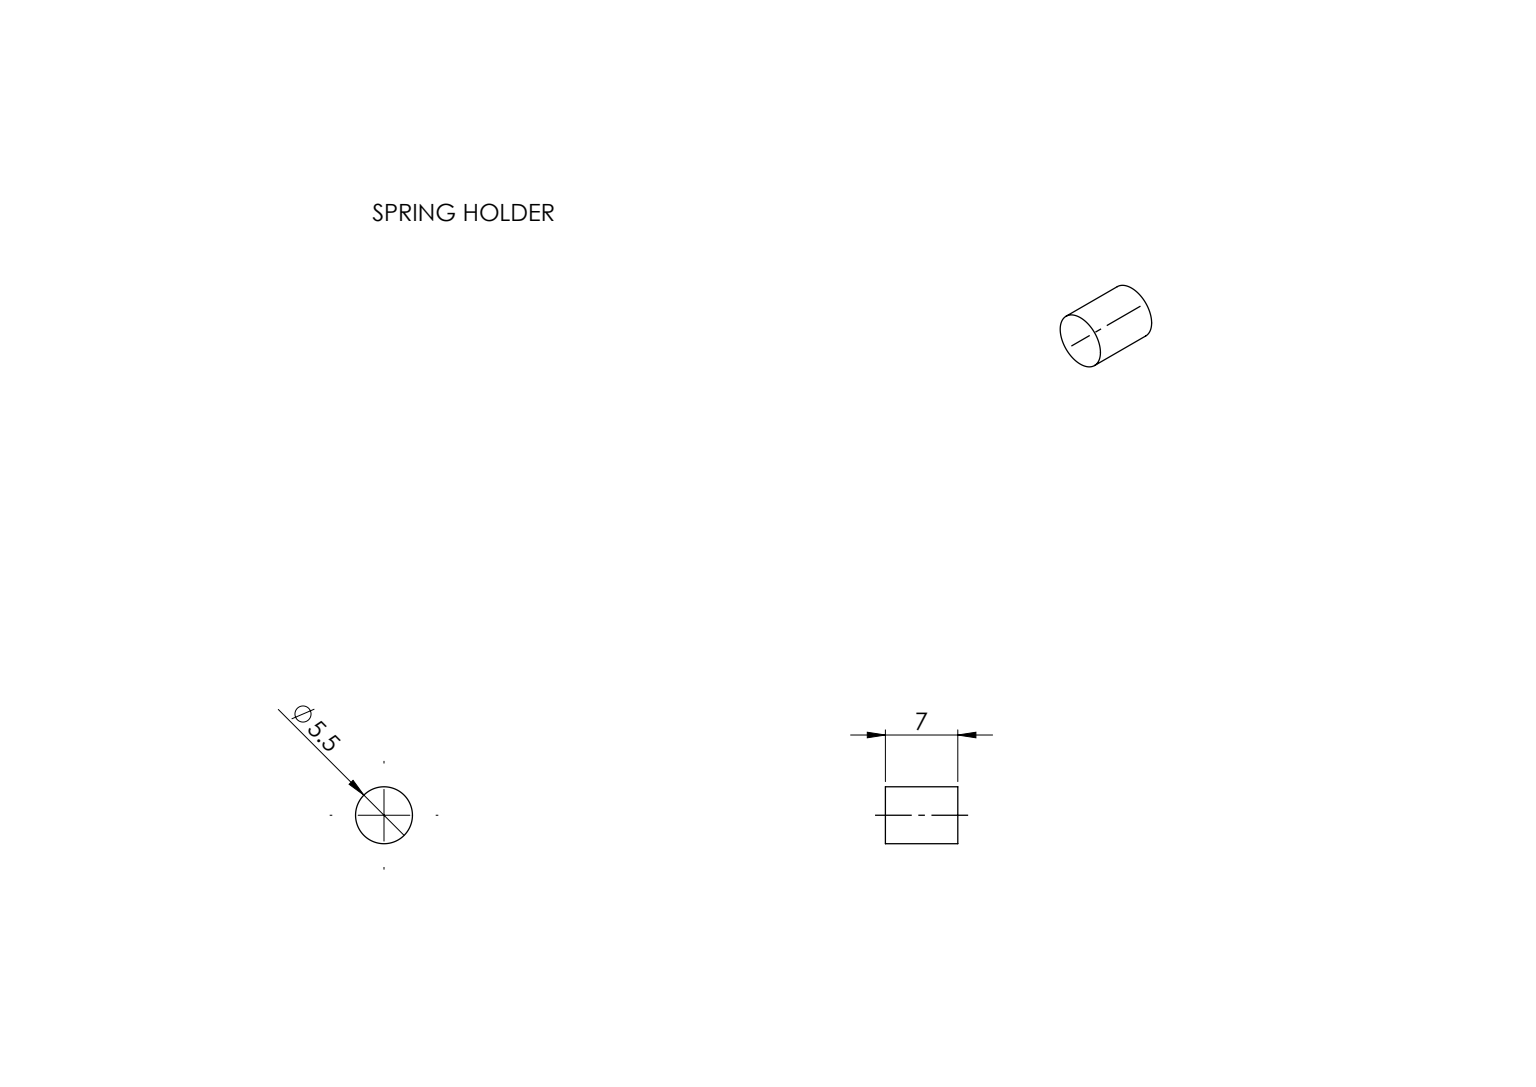
ISO-10303-21;
HEADER;
FILE_DESCRIPTION (('STEP AP214'),
    '1' );
FILE_NAME ('spring holder.step',
    '2026-10-05T05:16:24',
    ( '' ),
    ( '' ),
    'SwSTEP 2.0',
    'SolidWorks 2026',
    '' );
FILE_SCHEMA (( 'AUTOMOTIVE_DESIGN' ));
ENDSEC;

DATA;
#534=CARTESIAN_POINT ( 'NONE',  ( 1.653273178848927064E-15, -7.500000000000000000, 11.00000000000000178 ) ) ;
#1888=MECHANICAL_DESIGN_GEOMETRIC_PRESENTATION_REPRESENTATION('',(#79567),#65141);
#2272=UNCERTAINTY_MEASURE_WITH_UNIT (LENGTH_MEASURE( 1.000000000000000082E-05 ), #31200, 'distance_accuracy_value', 'NONE');
#3063=VERTEX_POINT ( 'NONE', #51324 ) ;
#4174=( LENGTH_UNIT ( ) NAMED_UNIT ( * ) SI_UNIT ( .MILLI., .METRE. ) );
#4325=VERTEX_POINT ( 'NONE', #12504 ) ;
#7485=DIRECTION ( 'NONE',  ( 1.000000000000000000, 0.000000000000000000, -0.000000000000000000 ) ) ;
#8165=AXIS2_PLACEMENT_3D ( 'NONE', #19814, #47277, #40542 ) ;
#8975=CARTESIAN_POINT ( 'NONE',  ( 1.653273178848927064E-15, -7.500000000000000000, 11.00000000000000178 ) ) ;
#9438=DIRECTION ( 'NONE',  ( 0.000000000000000000, 0.000000000000000000, 1.000000000000000000 ) ) ;
#10500=( NAMED_UNIT ( * ) SI_UNIT ( $, .STERADIAN. ) SOLID_ANGLE_UNIT ( ) );
#10751=VERTEX_POINT ( 'NONE', #18242 ) ;
#11381=( NAMED_UNIT ( * ) SI_UNIT ( $, .STERADIAN. ) SOLID_ANGLE_UNIT ( ) );
#11508=ORIENTED_EDGE ( 'NONE', *, *, #70839, .F. ) ;
#11527=SHAPE_REPRESENTATION ( 'spring holder', ( #83448 ), #56118 ) ;
#11836=FILL_AREA_STYLE ('',( #72187 ) ) ;
#12321=DIRECTION ( 'NONE',  ( 1.000000000000000000, 0.000000000000000000, -0.000000000000000000 ) ) ;
#12504=CARTESIAN_POINT ( 'NONE',  ( 2.750000000000001776, -7.500000000000000000, 11.00000000000000178 ) ) ;
#13007=APPLICATION_CONTEXT ( 'automotive_design' ) ;
#13034=CIRCLE ( 'NONE', #79184, 2.750000000000000000 ) ;
#13162=DIRECTION ( 'NONE',  ( 0.000000000000000000, 0.000000000000000000, 1.000000000000000000 ) ) ;
#13210=EDGE_LOOP ( 'NONE', ( #17041, #44560, #75203, #61413 ) ) ;
#14259=CARTESIAN_POINT ( 'NONE',  ( -2.749999999999998224, -7.500000000000000000, 11.00000000000000178 ) ) ;
#15733=DIRECTION ( 'NONE',  ( 0.000000000000000000, 0.000000000000000000, 1.000000000000000000 ) ) ;
#15761=DIRECTION ( 'NONE',  ( 1.000000000000000000, 0.000000000000000000, 0.000000000000000000 ) ) ;
#16170=DIRECTION ( 'NONE',  ( 0.000000000000000000, 0.000000000000000000, 1.000000000000000000 ) ) ;
#16194=CARTESIAN_POINT ( 'NONE',  ( 1.653273178848927064E-15, -7.500000000000000000, 11.00000000000000178 ) ) ;
#16800=PRESENTATION_STYLE_ASSIGNMENT (( #37969 ) ) ;
#17041=ORIENTED_EDGE ( 'NONE', *, *, #71531, .T. ) ;
#17272=COLOUR_RGB ( '', 0.66274510, 0.83137255, 0.94901961) ;
#17657=VECTOR ( 'NONE', #15733, 1000.000000000000000 ) ;
#18242=CARTESIAN_POINT ( 'NONE',  ( 2.750000000000001776, -7.500000000000000000, 18.00000000000000355 ) ) ;
#19513=CARTESIAN_POINT ( 'NONE',  ( 1.653273178848927064E-15, -7.500000000000000000, 11.00000000000000178 ) ) ;
#19678=ADVANCED_FACE ( 'NONE', ( #57151 ), #77863, .T. ) ;
#19814=CARTESIAN_POINT ( 'NONE',  ( 1.653273178848927064E-15, -7.500000000000000000, 11.00000000000000178 ) ) ;
#19995=PRODUCT_DEFINITION ( 'UNKNOWN', '', #54748, #85206 ) ;
#23003=( GEOMETRIC_REPRESENTATION_CONTEXT ( 3 ) GLOBAL_UNCERTAINTY_ASSIGNED_CONTEXT ( ( #2272 ) ) GLOBAL_UNIT_ASSIGNED_CONTEXT ( ( #31200, #65434, #11381 ) ) REPRESENTATION_CONTEXT ( 'NONE', 'WORKASPACE' ) );
#23878=ORIENTED_EDGE ( 'NONE', *, *, #58802, .T. ) ;
#24904=COLOUR_RGB ( '', 0.66274510, 0.83137255, 0.94901961) ;
#26814=SURFACE_STYLE_USAGE ( .BOTH. , #33125 ) ;
#26851=DIRECTION ( 'NONE',  ( 0.000000000000000000, 0.000000000000000000, 1.000000000000000000 ) ) ;
#28181=DIRECTION ( 'NONE',  ( 0.000000000000000000, 0.000000000000000000, 1.000000000000000000 ) ) ;
#29592=AXIS2_PLACEMENT_3D ( 'NONE', #61073, #26851, #60180 ) ;
#30303=ORIENTED_EDGE ( 'NONE', *, *, #35419, .T. ) ;
#31200=( LENGTH_UNIT ( ) NAMED_UNIT ( * ) SI_UNIT ( .MILLI., .METRE. ) );
#31566=EDGE_LOOP ( 'NONE', ( #79815, #45791 ) ) ;
#32575=AXIS2_PLACEMENT_3D ( 'NONE', #534, #13162, #80749 ) ;
#32871=VERTEX_POINT ( 'NONE', #59707 ) ;
#33125=SURFACE_SIDE_STYLE ('',( #61472 ) ) ;
#34939=PLANE ( 'NONE',  #68533 ) ;
#35307=DIRECTION ( 'NONE',  ( 1.000000000000000000, 0.000000000000000000, 0.000000000000000000 ) ) ;
#35419=EDGE_CURVE ( 'NONE', #10751, #3063, #72731, .T. ) ;
#35562=LINE ( 'NONE', #77424, #17657 ) ;
#36528=UNCERTAINTY_MEASURE_WITH_UNIT (LENGTH_MEASURE( 1.000000000000000082E-05 ), #4174, 'distance_accuracy_value', 'NONE');
#37969=SURFACE_STYLE_USAGE ( .BOTH. , #53246 ) ;
#39006=ADVANCED_FACE ( 'NONE', ( #60940 ), #74026, .F. ) ;
#39898=PRESENTATION_STYLE_ASSIGNMENT (( #26814 ) ) ;
#40542=DIRECTION ( 'NONE',  ( 1.000000000000000000, 0.000000000000000000, 0.000000000000000000 ) ) ;
#40780=( NAMED_UNIT ( * ) SI_UNIT ( $, .STERADIAN. ) SOLID_ANGLE_UNIT ( ) );
#40850=LINE ( 'NONE', #14259, #69938 ) ;
#41724=MECHANICAL_DESIGN_GEOMETRIC_PRESENTATION_REPRESENTATION('',(#80559),#23003);
#43632=DIRECTION ( 'NONE',  ( 1.000000000000000000, 0.000000000000000000, 0.000000000000000000 ) ) ;
#44254=( NAMED_UNIT ( * ) PLANE_ANGLE_UNIT ( ) SI_UNIT ( $, .RADIAN. ) );
#44325=CLOSED_SHELL ( 'NONE', ( #19678, #71875, #39006, #63524 ) ) ;
#44560=ORIENTED_EDGE ( 'NONE', *, *, #70839, .T. ) ;
#44894=ORIENTED_EDGE ( 'NONE', *, *, #81635, .T. ) ;
#45791=ORIENTED_EDGE ( 'NONE', *, *, #81635, .F. ) ;
#46002=PRODUCT_CONTEXT ( 'NONE', #13007, 'mechanical' ) ;
#46452=CIRCLE ( 'NONE', #85289, 2.750000000000000000 ) ;
#47277=DIRECTION ( 'NONE',  ( 0.000000000000000000, 0.000000000000000000, 1.000000000000000000 ) ) ;
#48901=CARTESIAN_POINT ( 'NONE',  ( 1.653273178848927064E-15, -7.500000000000000000, 18.00000000000000355 ) ) ;
#51324=CARTESIAN_POINT ( 'NONE',  ( -2.749999999999998224, -7.500000000000000000, 18.00000000000000355 ) ) ;
#53246=SURFACE_SIDE_STYLE ('',( #71740 ) ) ;
#53492=DIRECTION ( 'NONE',  ( 0.000000000000000000, 0.000000000000000000, 1.000000000000000000 ) ) ;
#53838=( NAMED_UNIT ( * ) PLANE_ANGLE_UNIT ( ) SI_UNIT ( $, .RADIAN. ) );
#54748=PRODUCT_DEFINITION_FORMATION_WITH_SPECIFIED_SOURCE ( 'ANY', '', #75728, .NOT_KNOWN. ) ;
#56118=( GEOMETRIC_REPRESENTATION_CONTEXT ( 3 ) GLOBAL_UNCERTAINTY_ASSIGNED_CONTEXT ( ( #36528 ) ) GLOBAL_UNIT_ASSIGNED_CONTEXT ( ( #4174, #44254, #10500 ) ) REPRESENTATION_CONTEXT ( 'NONE', 'WORKASPACE' ) );
#57151=FACE_OUTER_BOUND ( 'NONE', #13210, .T. ) ;
#57745=EDGE_LOOP ( 'NONE', ( #11508, #44894, #23878, #77482 ) ) ;
#58802=EDGE_CURVE ( 'NONE', #4325, #10751, #35562, .T. ) ;
#59139=EDGE_CURVE ( 'NONE', #3063, #10751, #46452, .T. ) ;
#59398=MANIFOLD_SOLID_BREP ( 'Boss-Extrude1', #44325 ) ;
#59707=CARTESIAN_POINT ( 'NONE',  ( -2.749999999999998224, -7.500000000000000000, 11.00000000000000178 ) ) ;
#60143=( LENGTH_UNIT ( ) NAMED_UNIT ( * ) SI_UNIT ( .MILLI., .METRE. ) );
#60180=DIRECTION ( 'NONE',  ( 1.000000000000000000, 0.000000000000000000, 0.000000000000000000 ) ) ;
#60940=FACE_OUTER_BOUND ( 'NONE', #31566, .T. ) ;
#61073=CARTESIAN_POINT ( 'NONE',  ( 1.653273178848927064E-15, -7.500000000000000000, 18.00000000000000355 ) ) ;
#61413=ORIENTED_EDGE ( 'NONE', *, *, #58802, .F. ) ;
#61472=SURFACE_STYLE_FILL_AREA ( #73683 ) ;
#62763=CARTESIAN_POINT ( 'NONE',  ( 0.000000000000000000, 0.000000000000000000, 0.000000000000000000 ) ) ;
#63524=ADVANCED_FACE ( 'NONE', ( #83142 ), #34939, .T. ) ;
#63534=EDGE_LOOP ( 'NONE', ( #30303, #80308 ) ) ;
#65141=( GEOMETRIC_REPRESENTATION_CONTEXT ( 3 ) GLOBAL_UNCERTAINTY_ASSIGNED_CONTEXT ( ( #77946 ) ) GLOBAL_UNIT_ASSIGNED_CONTEXT ( ( #60143, #53838, #40780 ) ) REPRESENTATION_CONTEXT ( 'NONE', 'WORKASPACE' ) );
#65434=( NAMED_UNIT ( * ) PLANE_ANGLE_UNIT ( ) SI_UNIT ( $, .RADIAN. ) );
#67802=FILL_AREA_STYLE_COLOUR ( '', #24904 ) ;
#68316=DIRECTION ( 'NONE',  ( 0.000000000000000000, 0.000000000000000000, 1.000000000000000000 ) ) ;
#68533=AXIS2_PLACEMENT_3D ( 'NONE', #48901, #28181, #7485 ) ;
#69938=VECTOR ( 'NONE', #68316, 1000.000000000000000 ) ;
#70839=EDGE_CURVE ( 'NONE', #32871, #3063, #40850, .T. ) ;
#71531=EDGE_CURVE ( 'NONE', #4325, #32871, #77199, .T. ) ;
#71649=APPLICATION_CONTEXT ( 'automotive_design' ) ;
#71740=SURFACE_STYLE_FILL_AREA ( #11836 ) ;
#71875=ADVANCED_FACE ( 'NONE', ( #86054 ), #79298, .T. ) ;
#72187=FILL_AREA_STYLE_COLOUR ( '', #17272 ) ;
#72671=AXIS2_PLACEMENT_3D ( 'NONE', #8975, #16170, #43632 ) ;
#72731=CIRCLE ( 'NONE', #29592, 2.750000000000000000 ) ;
#73683=FILL_AREA_STYLE ('',( #67802 ) ) ;
#74026=PLANE ( 'NONE',  #88832 ) ;
#74442=PRODUCT_DEFINITION_SHAPE ( 'NONE', 'NONE',  #19995 ) ;
#75203=ORIENTED_EDGE ( 'NONE', *, *, #35419, .F. ) ;
#75728=PRODUCT ( 'spring holder', 'spring holder', '', ( #46002 ) ) ;
#77199=CIRCLE ( 'NONE', #32575, 2.750000000000000000 ) ;
#77424=CARTESIAN_POINT ( 'NONE',  ( 2.750000000000001776, -7.500000000000000000, 11.00000000000000178 ) ) ;
#77482=ORIENTED_EDGE ( 'NONE', *, *, #59139, .F. ) ;
#77863=CYLINDRICAL_SURFACE ( 'NONE', #72671, 2.750000000000000000 ) ;
#77946=UNCERTAINTY_MEASURE_WITH_UNIT (LENGTH_MEASURE( 1.000000000000000082E-05 ), #60143, 'distance_accuracy_value', 'NONE');
#79184=AXIS2_PLACEMENT_3D ( 'NONE', #16194, #9438, #15761 ) ;
#79298=CYLINDRICAL_SURFACE ( 'NONE', #8165, 2.750000000000000000 ) ;
#79567=STYLED_ITEM ( 'NONE', ( #39898 ), #59398 ) ;
#79815=ORIENTED_EDGE ( 'NONE', *, *, #71531, .F. ) ;
#80295=SHAPE_REPRESENTATION_RELATIONSHIP ( 'NONE' , 'NONE' ,  #11527, #83739 ) ;
#80308=ORIENTED_EDGE ( 'NONE', *, *, #59139, .T. ) ;
#80559=STYLED_ITEM ( 'NONE', ( #16800 ), #83739 ) ;
#80749=DIRECTION ( 'NONE',  ( 1.000000000000000000, 0.000000000000000000, 0.000000000000000000 ) ) ;
#80989=DIRECTION ( 'NONE',  ( 1.000000000000000000, 0.000000000000000000, 0.000000000000000000 ) ) ;
#81635=EDGE_CURVE ( 'NONE', #32871, #4325, #13034, .T. ) ;
#82112=DIRECTION ( 'NONE',  ( 0.000000000000000000, 0.000000000000000000, 1.000000000000000000 ) ) ;
#83142=FACE_OUTER_BOUND ( 'NONE', #63534, .T. ) ;
#83448=AXIS2_PLACEMENT_3D ( 'NONE', #62763, #83959, #35307 ) ;
#83739=ADVANCED_BREP_SHAPE_REPRESENTATION ( '', ( #59398, #83448 ), #56118 ) ;
#83959=DIRECTION ( 'NONE',  ( 0.000000000000000000, 0.000000000000000000, 1.000000000000000000 ) ) ;
#85206=PRODUCT_DEFINITION_CONTEXT ( 'detailed design', #71649, 'design' ) ;
#85289=AXIS2_PLACEMENT_3D ( 'NONE', #89088, #53492, #80989 ) ;
#86054=FACE_OUTER_BOUND ( 'NONE', #57745, .T. ) ;
#86569=SHAPE_DEFINITION_REPRESENTATION ( #74442, #11527 ) ;
#88832=AXIS2_PLACEMENT_3D ( 'NONE', #19513, #82112, #12321 ) ;
#89088=CARTESIAN_POINT ( 'NONE',  ( 1.653273178848927064E-15, -7.500000000000000000, 18.00000000000000355 ) ) ;
ENDSEC;
END-ISO-10303-21;
